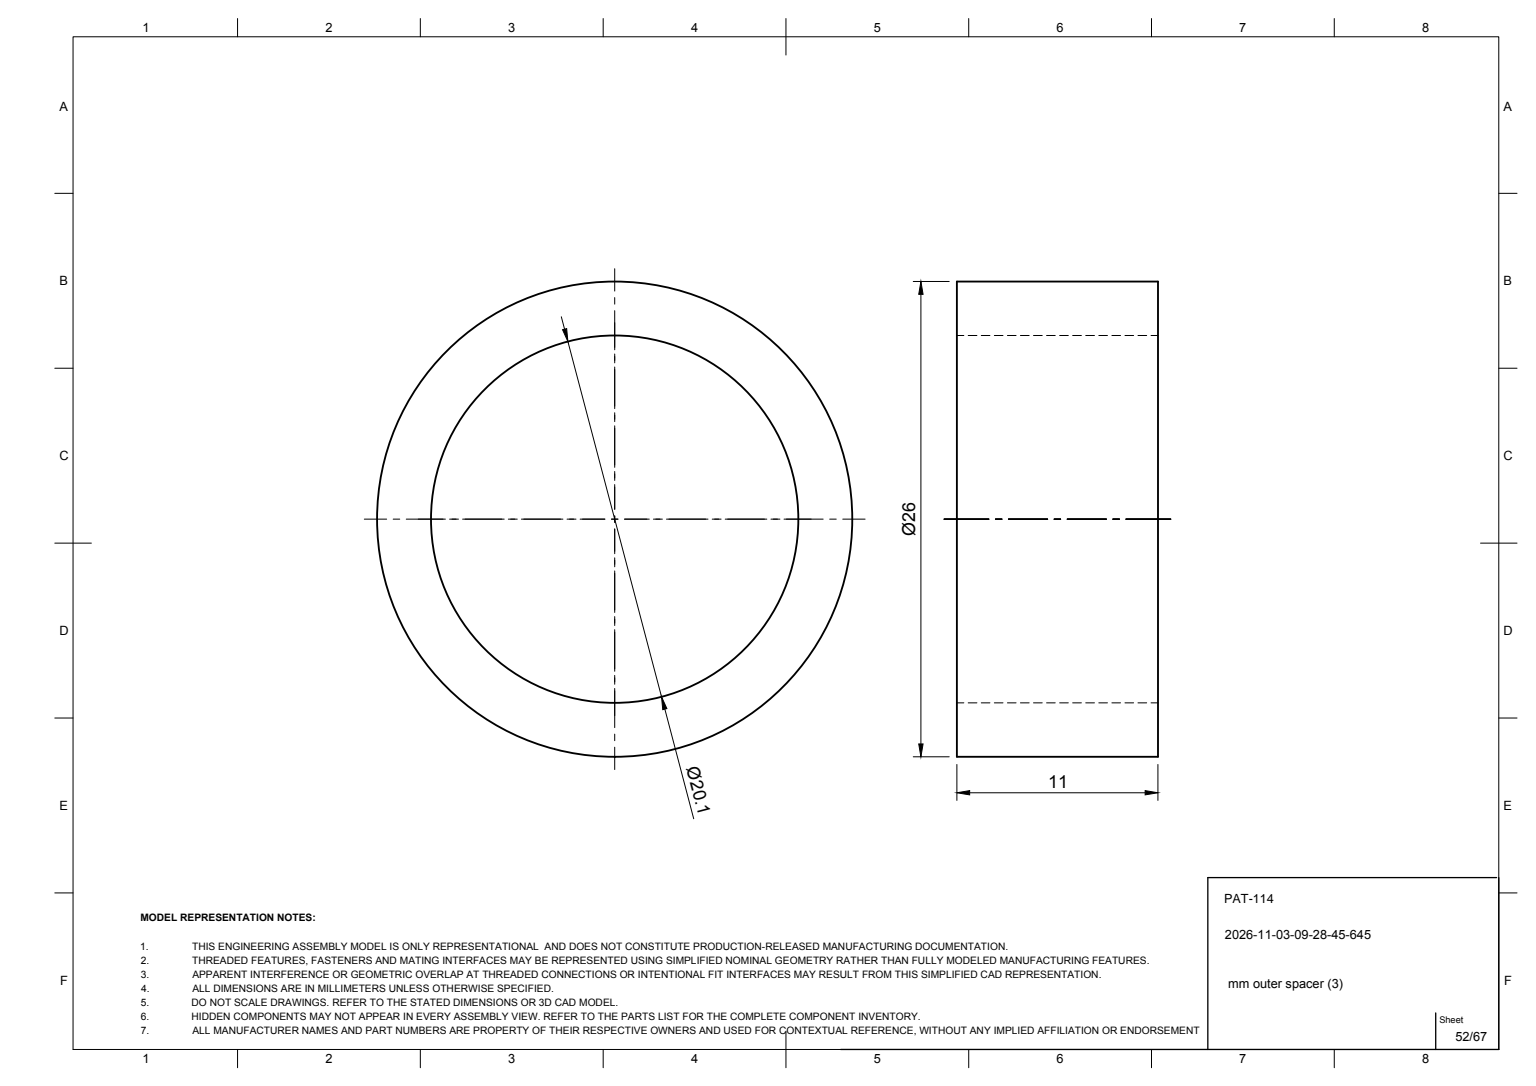
ISO-10303-21;
HEADER;
/* Generated by software containing ST-Developer
 * from STEP Tools, Inc. (www.steptools.com) 
 */

FILE_DESCRIPTION(
/* description */ ('Two-stage gear reducer in split housing'),
/* implementation_level */ '2;1');

FILE_NAME(
/* name */ 'mm outer spacer (3).step',
/* time_stamp */ '2026-10-28T03:22:31-07:00',
/* author */ (''),
/* organization */ (''),
/* preprocessor_version */ 'ST-DEVELOPER v20.2',
/* originating_system */ 'Autodesk Translation Framework v15.17.0.0',
/* authorisation */ '');

FILE_SCHEMA (('AUTOMOTIVE_DESIGN { 1 0 10303 214 3 1 1 }'));
ENDSEC;

DATA;
#10=MECHANICAL_DESIGN_GEOMETRIC_PRESENTATION_REPRESENTATION('',(#1290),#73366);
#1163=SHAPE_REPRESENTATION_RELATIONSHIP('SRR','None',#73654,#1219);
#1219=ADVANCED_BREP_SHAPE_REPRESENTATION('',(#1359),#73350);
#1290=STYLED_ITEM('',(#73974),#1359);
#1359=MANIFOLD_SOLID_BREP('Body1',#16180);
#1570=FACE_BOUND('',#3695,.T.);
#1571=FACE_BOUND('',#3697,.T.);
#1880=PLANE('',#18015);
#1881=PLANE('',#18016);
#2583=FACE_OUTER_BOUND('',#3692,.T.);
#2584=FACE_OUTER_BOUND('',#3693,.T.);
#2585=FACE_OUTER_BOUND('',#3694,.T.);
#2586=FACE_OUTER_BOUND('',#3696,.T.);
#3692=EDGE_LOOP('',(#13119,#13120,#13121,#13122));
#3693=EDGE_LOOP('',(#13123,#13124,#13125,#13126));
#3694=EDGE_LOOP('',(#13127));
#3695=EDGE_LOOP('',(#13128));
#3696=EDGE_LOOP('',(#13129));
#3697=EDGE_LOOP('',(#13130));
#4696=LINE('',#37606,#5720);
#4697=LINE('',#37612,#5721);
#5720=VECTOR('',#21496,1.005);
#5721=VECTOR('',#21503,1.3);
#6642=CIRCLE('',#18010,1.005);
#6643=CIRCLE('',#18011,1.005);
#6644=CIRCLE('',#18013,1.3);
#6645=CIRCLE('',#18014,1.3);
#7711=VERTEX_POINT('',#37603);
#7712=VERTEX_POINT('',#37605);
#7713=VERTEX_POINT('',#37609);
#7714=VERTEX_POINT('',#37611);
#9613=EDGE_CURVE('',#7711,#7711,#6642,.T.);
#9614=EDGE_CURVE('',#7711,#7712,#4696,.T.);
#9615=EDGE_CURVE('',#7712,#7712,#6643,.T.);
#9616=EDGE_CURVE('',#7713,#7713,#6644,.T.);
#9617=EDGE_CURVE('',#7713,#7714,#4697,.T.);
#9618=EDGE_CURVE('',#7714,#7714,#6645,.T.);
#13119=ORIENTED_EDGE('',*,*,#9613,.F.);
#13120=ORIENTED_EDGE('',*,*,#9614,.T.);
#13121=ORIENTED_EDGE('',*,*,#9615,.T.);
#13122=ORIENTED_EDGE('',*,*,#9614,.F.);
#13123=ORIENTED_EDGE('',*,*,#9616,.F.);
#13124=ORIENTED_EDGE('',*,*,#9617,.T.);
#13125=ORIENTED_EDGE('',*,*,#9618,.T.);
#13126=ORIENTED_EDGE('',*,*,#9617,.F.);
#13127=ORIENTED_EDGE('',*,*,#9616,.T.);
#13128=ORIENTED_EDGE('',*,*,#9613,.T.);
#13129=ORIENTED_EDGE('',*,*,#9618,.F.);
#13130=ORIENTED_EDGE('',*,*,#9615,.F.);
#15121=CYLINDRICAL_SURFACE('',#18009,1.005);
#15122=CYLINDRICAL_SURFACE('',#18012,1.3);
#15790=ADVANCED_FACE('',(#2583),#15121,.F.);
#15791=ADVANCED_FACE('',(#2584),#15122,.T.);
#15792=ADVANCED_FACE('',(#2585,#1570),#1880,.T.);
#15793=ADVANCED_FACE('',(#2586,#1571),#1881,.F.);
#16180=CLOSED_SHELL('',(#15790,#15791,#15792,#15793));
#18008=AXIS2_PLACEMENT_3D('',#37601,#21490,#21491);
#18009=AXIS2_PLACEMENT_3D('',#37602,#21492,#21493);
#18010=AXIS2_PLACEMENT_3D('',#37604,#21494,#21495);
#18011=AXIS2_PLACEMENT_3D('',#37607,#21497,#21498);
#18012=AXIS2_PLACEMENT_3D('',#37608,#21499,#21500);
#18013=AXIS2_PLACEMENT_3D('',#37610,#21501,#21502);
#18014=AXIS2_PLACEMENT_3D('',#37613,#21504,#21505);
#18015=AXIS2_PLACEMENT_3D('',#37614,#21506,#21507);
#18016=AXIS2_PLACEMENT_3D('',#37615,#21508,#21509);
#21490=DIRECTION('axis',(0.,0.,1.));
#21491=DIRECTION('refdir',(1.,0.,0.));
#21492=DIRECTION('center_axis',(0.,1.,0.));
#21493=DIRECTION('ref_axis',(1.,0.,0.));
#21494=DIRECTION('center_axis',(0.,-1.,0.));
#21495=DIRECTION('ref_axis',(1.,0.,0.));
#21496=DIRECTION('',(0.,-1.,0.));
#21497=DIRECTION('center_axis',(0.,-1.,0.));
#21498=DIRECTION('ref_axis',(1.,0.,0.));
#21499=DIRECTION('center_axis',(0.,1.,0.));
#21500=DIRECTION('ref_axis',(1.,0.,0.));
#21501=DIRECTION('center_axis',(0.,1.,0.));
#21502=DIRECTION('ref_axis',(1.,0.,0.));
#21503=DIRECTION('',(0.,-1.,0.));
#21504=DIRECTION('center_axis',(0.,1.,0.));
#21505=DIRECTION('ref_axis',(1.,0.,0.));
#21506=DIRECTION('center_axis',(0.,1.,0.));
#21507=DIRECTION('ref_axis',(1.,0.,0.));
#21508=DIRECTION('center_axis',(0.,1.,0.));
#21509=DIRECTION('ref_axis',(1.,0.,0.));
#37601=CARTESIAN_POINT('',(0.,0.,0.));
#37602=CARTESIAN_POINT('Origin',(6.,6.7,10.));
#37603=CARTESIAN_POINT('',(4.995,7.8,10.));
#37604=CARTESIAN_POINT('Origin',(6.,7.8,10.));
#37605=CARTESIAN_POINT('',(4.995,6.7,10.));
#37606=CARTESIAN_POINT('',(4.995,6.7,10.));
#37607=CARTESIAN_POINT('Origin',(6.,6.7,10.));
#37608=CARTESIAN_POINT('Origin',(6.,6.7,10.));
#37609=CARTESIAN_POINT('',(4.7,7.8,10.));
#37610=CARTESIAN_POINT('Origin',(6.,7.8,10.));
#37611=CARTESIAN_POINT('',(4.7,6.7,10.));
#37612=CARTESIAN_POINT('',(4.7,6.7,10.));
#37613=CARTESIAN_POINT('Origin',(6.,6.7,10.));
#37614=CARTESIAN_POINT('Origin',(6.,7.8,10.));
#37615=CARTESIAN_POINT('Origin',(6.,6.7,10.));
#73286=UNCERTAINTY_MEASURE_WITH_UNIT(LENGTH_MEASURE(0.001),#73367,
'DISTANCE_ACCURACY_VALUE',
'Maximum model space distance between geometric entities at asserted c
onnectivities');
#73302=UNCERTAINTY_MEASURE_WITH_UNIT(LENGTH_MEASURE(0.001),#73367,
'DISTANCE_ACCURACY_VALUE',
'Maximum model space distance between geometric entities at asserted c
onnectivities');
#73350=(
GEOMETRIC_REPRESENTATION_CONTEXT(3)
GLOBAL_UNCERTAINTY_ASSIGNED_CONTEXT((#73286))
GLOBAL_UNIT_ASSIGNED_CONTEXT((#73367,#73369,#73370))
REPRESENTATION_CONTEXT('','3D')
);
#73366=(
GEOMETRIC_REPRESENTATION_CONTEXT(3)
GLOBAL_UNCERTAINTY_ASSIGNED_CONTEXT((#73302))
GLOBAL_UNIT_ASSIGNED_CONTEXT((#73367,#73369,#73370))
REPRESENTATION_CONTEXT('','3D')
);
#73367=(
LENGTH_UNIT()
NAMED_UNIT(*)
SI_UNIT(.CENTI.,.METRE.)
);
#73369=(
NAMED_UNIT(*)
PLANE_ANGLE_UNIT()
SI_UNIT($,.RADIAN.)
);
#73370=(
NAMED_UNIT(*)
SI_UNIT($,.STERADIAN.)
SOLID_ANGLE_UNIT()
);
#73418=SHAPE_DEFINITION_REPRESENTATION(#73551,#73654);
#73551=PRODUCT_DEFINITION_SHAPE('',$,#73718);
#73654=SHAPE_REPRESENTATION('',(#18008),#73350);
#73670=PRODUCT_DEFINITION_CONTEXT('part definition',#73861,'design');
#73718=PRODUCT_DEFINITION('mm outer spacer (3)','mm outer spacer (3)',#73781,
#73670);
#73781=PRODUCT_DEFINITION_FORMATION('',$,#73910);
#73861=APPLICATION_CONTEXT(
'Core Data for Automotive Mechanical Design Process');
#73862=PRODUCT_CONTEXT('part definition',#73861,'mechanical');
#73910=PRODUCT('mm outer spacer (3)','mm outer spacer (3)',
'mm outer spacer (3)',(#73862));
#73968=COLOUR_RGB('Light Blue',0.38,0.62,0.78);
#73969=FILL_AREA_STYLE_COLOUR('',#73968);
#73970=FILL_AREA_STYLE('',(#73969));
#73971=SURFACE_STYLE_FILL_AREA(#73970);
#73972=SURFACE_SIDE_STYLE('',(#73971));
#73973=SURFACE_STYLE_USAGE(.BOTH.,#73972);
#73974=PRESENTATION_STYLE_ASSIGNMENT((#73973));
ENDSEC;
END-ISO-10303-21;
